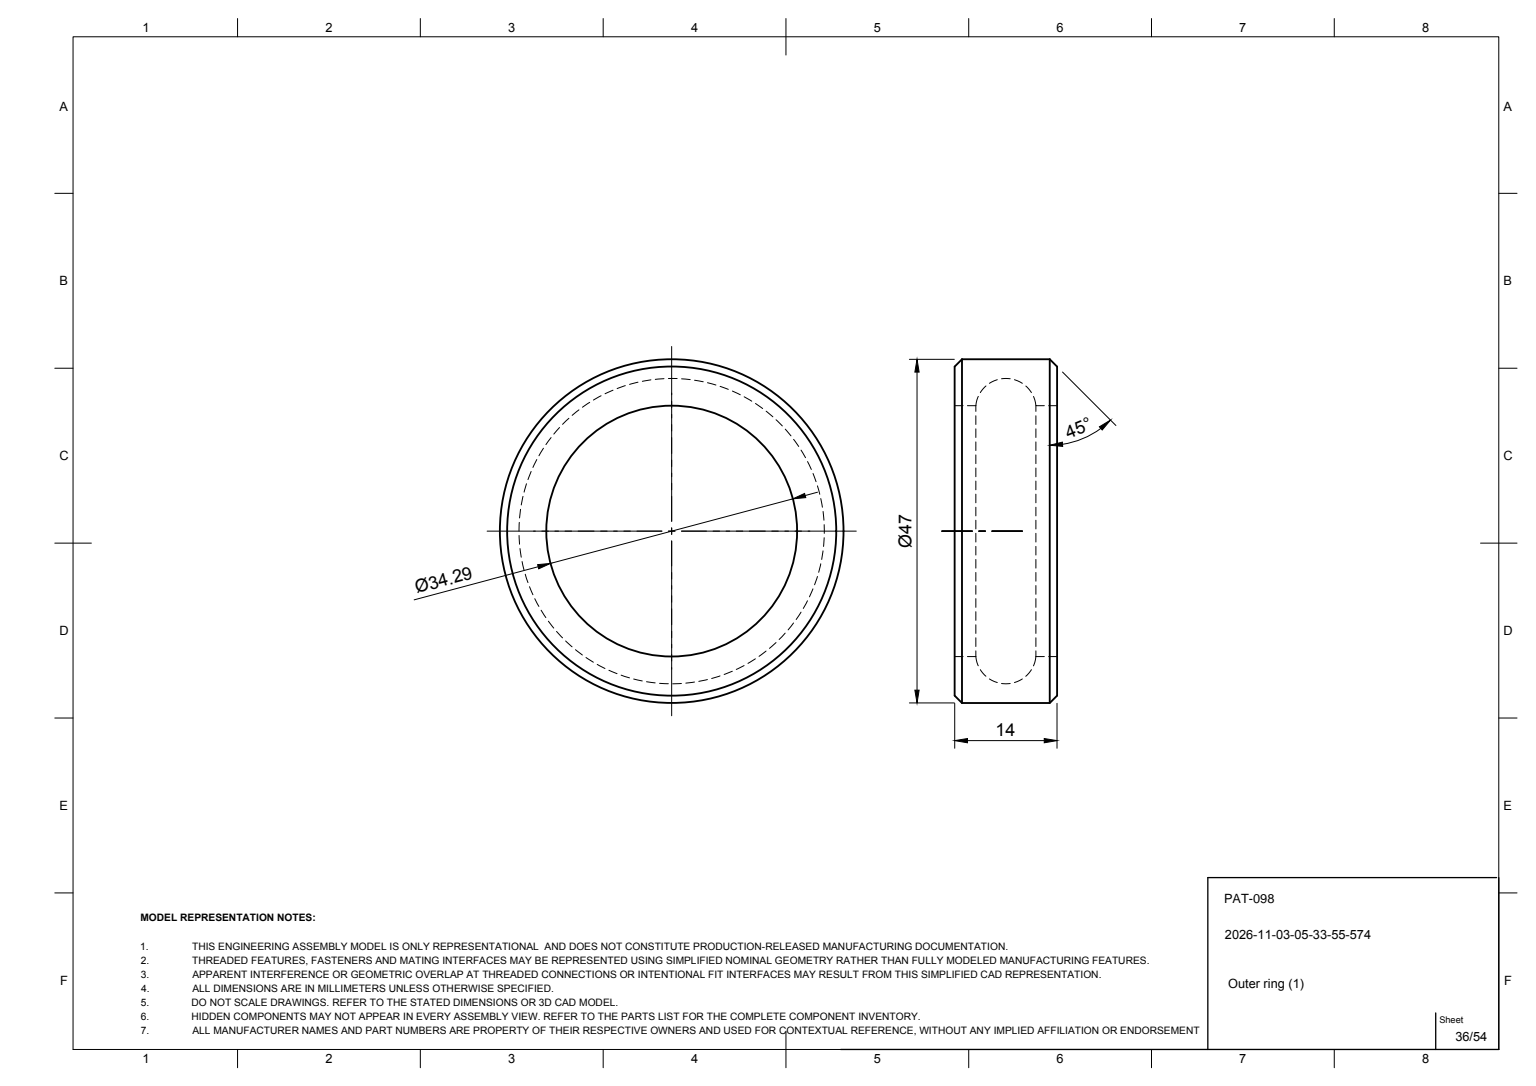
ISO-10303-21;
HEADER;
/* Generated by software containing ST-Developer
 * from STEP Tools, Inc. (www.steptools.com) 
 */

FILE_DESCRIPTION(
/* description */ ('Spring compression tester'),
/* implementation_level */ '2;1');

FILE_NAME(
/* name */ 'Outer ring (1).step',
/* time_stamp */ '2026-10-28T03:24:11-07:00',
/* author */ (''),
/* organization */ (''),
/* preprocessor_version */ 'ST-DEVELOPER v20.2',
/* originating_system */ 'Autodesk Translation Framework v15.17.0.0',
/* authorisation */ '');

FILE_SCHEMA (('AUTOMOTIVE_DESIGN { 1 0 10303 214 3 1 1 }'));
ENDSEC;

DATA;
#10=MECHANICAL_DESIGN_GEOMETRIC_PRESENTATION_REPRESENTATION('',(#1140),#43521);
#930=TOROIDAL_SURFACE('',#20142,1.675,0.412776);
#956=CONICAL_SURFACE('',#20153,2.3,0.785398163397449);
#957=CONICAL_SURFACE('',#20157,2.3,0.785398163397449);
#1013=SHAPE_REPRESENTATION_RELATIONSHIP('SRR','None',#43827,#1073);
#1073=ADVANCED_BREP_SHAPE_REPRESENTATION('',(#1214),#43487);
#1140=STYLED_ITEM('',(#44202),#1214);
#1214=MANIFOLD_SOLID_BREP('Body1',#18578);
#1461=FACE_BOUND('',#3916,.T.);
#1462=FACE_BOUND('',#3921,.T.);
#1906=PLANE('',#20150);
#1907=PLANE('',#20159);
#2652=FACE_OUTER_BOUND('',#3913,.T.);
#2653=FACE_OUTER_BOUND('',#3914,.T.);
#2654=FACE_OUTER_BOUND('',#3915,.T.);
#2655=FACE_OUTER_BOUND('',#3917,.T.);
#2656=FACE_OUTER_BOUND('',#3918,.T.);
#2657=FACE_OUTER_BOUND('',#3919,.T.);
#2658=FACE_OUTER_BOUND('',#3920,.T.);
#2659=FACE_OUTER_BOUND('',#3922,.T.);
#3913=EDGE_LOOP('',(#14351,#14352,#14353,#14354,#14355,#14356));
#3914=EDGE_LOOP('',(#14357,#14358,#14359,#14360,#14361));
#3915=EDGE_LOOP('',(#14362));
#3916=EDGE_LOOP('',(#14363));
#3917=EDGE_LOOP('',(#14364,#14365,#14366,#14367));
#3918=EDGE_LOOP('',(#14368,#14369,#14370,#14371));
#3919=EDGE_LOOP('',(#14372,#14373,#14374,#14375));
#3920=EDGE_LOOP('',(#14376));
#3921=EDGE_LOOP('',(#14377));
#3922=EDGE_LOOP('',(#14378,#14379,#14380,#14381,#14382));
#5322=LINE('',#29064,#6754);
#5323=LINE('',#29073,#6755);
#5324=LINE('',#29077,#6756);
#5325=LINE('',#29081,#6757);
#5326=LINE('',#29084,#6758);
#6754=VECTOR('',#23644,1.71469);
#6755=VECTOR('',#23655,2.3);
#6756=VECTOR('',#23660,2.35);
#6757=VECTOR('',#23665,2.3);
#6758=VECTOR('',#23670,1.71469);
#7807=CIRCLE('',#20143,1.71469);
#7808=CIRCLE('',#20144,1.71469);
#7809=CIRCLE('',#20145,0.412776);
#7810=CIRCLE('',#20146,1.71469);
#7811=CIRCLE('',#20147,1.71469);
#7812=CIRCLE('',#20149,1.71469);
#7813=CIRCLE('',#20151,2.25);
#7814=CIRCLE('',#20152,1.71469);
#7815=CIRCLE('',#20154,2.35);
#7816=CIRCLE('',#20156,2.35);
#7817=CIRCLE('',#20158,2.25);
#8853=VERTEX_POINT('',#29052);
#8854=VERTEX_POINT('',#29053);
#8855=VERTEX_POINT('',#29056);
#8856=VERTEX_POINT('',#29058);
#8857=VERTEX_POINT('',#29062);
#8858=VERTEX_POINT('',#29066);
#8859=VERTEX_POINT('',#29068);
#8860=VERTEX_POINT('',#29071);
#8861=VERTEX_POINT('',#29075);
#8862=VERTEX_POINT('',#29079);
#10840=EDGE_CURVE('',#8853,#8854,#7807,.T.);
#10841=EDGE_CURVE('',#8854,#8853,#7808,.T.);
#10842=EDGE_CURVE('',#8854,#8855,#7809,.T.);
#10843=EDGE_CURVE('',#8856,#8855,#7810,.T.);
#10844=EDGE_CURVE('',#8855,#8856,#7811,.T.);
#10845=EDGE_CURVE('',#8857,#8857,#7812,.T.);
#10846=EDGE_CURVE('',#8857,#8856,#5322,.T.);
#10847=EDGE_CURVE('',#8858,#8858,#7813,.T.);
#10848=EDGE_CURVE('',#8859,#8859,#7814,.T.);
#10849=EDGE_CURVE('',#8860,#8860,#7815,.T.);
#10850=EDGE_CURVE('',#8860,#8858,#5323,.T.);
#10851=EDGE_CURVE('',#8861,#8861,#7816,.T.);
#10852=EDGE_CURVE('',#8861,#8860,#5324,.T.);
#10853=EDGE_CURVE('',#8862,#8862,#7817,.T.);
#10854=EDGE_CURVE('',#8862,#8861,#5325,.T.);
#10855=EDGE_CURVE('',#8853,#8859,#5326,.T.);
#14351=ORIENTED_EDGE('',*,*,#10840,.F.);
#14352=ORIENTED_EDGE('',*,*,#10841,.F.);
#14353=ORIENTED_EDGE('',*,*,#10842,.T.);
#14354=ORIENTED_EDGE('',*,*,#10843,.F.);
#14355=ORIENTED_EDGE('',*,*,#10844,.F.);
#14356=ORIENTED_EDGE('',*,*,#10842,.F.);
#14357=ORIENTED_EDGE('',*,*,#10845,.T.);
#14358=ORIENTED_EDGE('',*,*,#10846,.T.);
#14359=ORIENTED_EDGE('',*,*,#10843,.T.);
#14360=ORIENTED_EDGE('',*,*,#10844,.T.);
#14361=ORIENTED_EDGE('',*,*,#10846,.F.);
#14362=ORIENTED_EDGE('',*,*,#10847,.F.);
#14363=ORIENTED_EDGE('',*,*,#10848,.T.);
#14364=ORIENTED_EDGE('',*,*,#10849,.F.);
#14365=ORIENTED_EDGE('',*,*,#10850,.T.);
#14366=ORIENTED_EDGE('',*,*,#10847,.T.);
#14367=ORIENTED_EDGE('',*,*,#10850,.F.);
#14368=ORIENTED_EDGE('',*,*,#10851,.F.);
#14369=ORIENTED_EDGE('',*,*,#10852,.T.);
#14370=ORIENTED_EDGE('',*,*,#10849,.T.);
#14371=ORIENTED_EDGE('',*,*,#10852,.F.);
#14372=ORIENTED_EDGE('',*,*,#10853,.F.);
#14373=ORIENTED_EDGE('',*,*,#10854,.T.);
#14374=ORIENTED_EDGE('',*,*,#10851,.T.);
#14375=ORIENTED_EDGE('',*,*,#10854,.F.);
#14376=ORIENTED_EDGE('',*,*,#10853,.T.);
#14377=ORIENTED_EDGE('',*,*,#10845,.F.);
#14378=ORIENTED_EDGE('',*,*,#10840,.T.);
#14379=ORIENTED_EDGE('',*,*,#10841,.T.);
#14380=ORIENTED_EDGE('',*,*,#10855,.T.);
#14381=ORIENTED_EDGE('',*,*,#10848,.F.);
#14382=ORIENTED_EDGE('',*,*,#10855,.F.);
#17242=CYLINDRICAL_SURFACE('',#20148,1.71469);
#17243=CYLINDRICAL_SURFACE('',#20155,2.35);
#17244=CYLINDRICAL_SURFACE('',#20160,1.71469);
#17976=ADVANCED_FACE('',(#2652),#930,.F.);
#17977=ADVANCED_FACE('',(#2653),#17242,.F.);
#17978=ADVANCED_FACE('',(#2654,#1461),#1906,.T.);
#17979=ADVANCED_FACE('',(#2655),#956,.T.);
#17980=ADVANCED_FACE('',(#2656),#17243,.T.);
#17981=ADVANCED_FACE('',(#2657),#957,.T.);
#17982=ADVANCED_FACE('',(#2658,#1462),#1907,.T.);
#17983=ADVANCED_FACE('',(#2659),#17244,.F.);
#18578=CLOSED_SHELL('',(#17976,#17977,#17978,#17979,#17980,#17981,#17982,
#17983));
#20141=AXIS2_PLACEMENT_3D('',#29050,#23626,#23627);
#20142=AXIS2_PLACEMENT_3D('',#29051,#23628,#23629);
#20143=AXIS2_PLACEMENT_3D('',#29054,#23630,#23631);
#20144=AXIS2_PLACEMENT_3D('',#29055,#23632,#23633);
#20145=AXIS2_PLACEMENT_3D('',#29057,#23634,#23635);
#20146=AXIS2_PLACEMENT_3D('',#29059,#23636,#23637);
#20147=AXIS2_PLACEMENT_3D('',#29060,#23638,#23639);
#20148=AXIS2_PLACEMENT_3D('',#29061,#23640,#23641);
#20149=AXIS2_PLACEMENT_3D('',#29063,#23642,#23643);
#20150=AXIS2_PLACEMENT_3D('',#29065,#23645,#23646);
#20151=AXIS2_PLACEMENT_3D('',#29067,#23647,#23648);
#20152=AXIS2_PLACEMENT_3D('',#29069,#23649,#23650);
#20153=AXIS2_PLACEMENT_3D('',#29070,#23651,#23652);
#20154=AXIS2_PLACEMENT_3D('',#29072,#23653,#23654);
#20155=AXIS2_PLACEMENT_3D('',#29074,#23656,#23657);
#20156=AXIS2_PLACEMENT_3D('',#29076,#23658,#23659);
#20157=AXIS2_PLACEMENT_3D('',#29078,#23661,#23662);
#20158=AXIS2_PLACEMENT_3D('',#29080,#23663,#23664);
#20159=AXIS2_PLACEMENT_3D('',#29082,#23666,#23667);
#20160=AXIS2_PLACEMENT_3D('',#29083,#23668,#23669);
#23626=DIRECTION('axis',(0.,0.,1.));
#23627=DIRECTION('refdir',(1.,0.,0.));
#23628=DIRECTION('center_axis',(0.,-1.,0.));
#23629=DIRECTION('ref_axis',(0.,0.,-1.));
#23630=DIRECTION('center_axis',(0.,-1.,0.));
#23631=DIRECTION('ref_axis',(1.,0.,0.));
#23632=DIRECTION('center_axis',(0.,-1.,0.));
#23633=DIRECTION('ref_axis',(1.,0.,0.));
#23634=DIRECTION('center_axis',(1.,0.,1.22464679914735E-16));
#23635=DIRECTION('ref_axis',(-1.22464679914735E-16,0.,1.));
#23636=DIRECTION('center_axis',(0.,1.,0.));
#23637=DIRECTION('ref_axis',(1.,0.,0.));
#23638=DIRECTION('center_axis',(0.,1.,0.));
#23639=DIRECTION('ref_axis',(1.,0.,0.));
#23640=DIRECTION('center_axis',(0.,-1.,0.));
#23641=DIRECTION('ref_axis',(1.,0.,0.));
#23642=DIRECTION('center_axis',(0.,-1.,0.));
#23643=DIRECTION('ref_axis',(1.,0.,0.));
#23644=DIRECTION('',(0.,1.,0.));
#23645=DIRECTION('center_axis',(0.,1.,0.));
#23646=DIRECTION('ref_axis',(0.,0.,1.));
#23647=DIRECTION('center_axis',(0.,-1.,0.));
#23648=DIRECTION('ref_axis',(1.,0.,0.));
#23649=DIRECTION('center_axis',(0.,-1.,0.));
#23650=DIRECTION('ref_axis',(1.,0.,0.));
#23651=DIRECTION('center_axis',(0.,-1.,0.));
#23652=DIRECTION('ref_axis',(1.,0.,0.));
#23653=DIRECTION('center_axis',(0.,-1.,0.));
#23654=DIRECTION('ref_axis',(1.,0.,0.));
#23655=DIRECTION('',(0.707106781186548,0.707106781186547,8.65956056235494E-17));
#23656=DIRECTION('center_axis',(0.,-1.,0.));
#23657=DIRECTION('ref_axis',(1.,0.,0.));
#23658=DIRECTION('center_axis',(0.,-1.,0.));
#23659=DIRECTION('ref_axis',(1.,0.,0.));
#23660=DIRECTION('',(0.,1.,0.));
#23661=DIRECTION('center_axis',(0.,1.,0.));
#23662=DIRECTION('ref_axis',(1.,0.,0.));
#23663=DIRECTION('center_axis',(0.,-1.,0.));
#23664=DIRECTION('ref_axis',(1.,0.,0.));
#23665=DIRECTION('',(-0.707106781186548,0.707106781186547,-8.65956056235494E-17));
#23666=DIRECTION('center_axis',(0.,-1.,0.));
#23667=DIRECTION('ref_axis',(0.,0.,-1.));
#23668=DIRECTION('center_axis',(0.,-1.,0.));
#23669=DIRECTION('ref_axis',(1.,0.,0.));
#23670=DIRECTION('',(0.,1.,0.));
#29050=CARTESIAN_POINT('',(0.,0.,0.));
#29051=CARTESIAN_POINT('Origin',(0.,0.,0.));
#29052=CARTESIAN_POINT('',(-1.71469,0.410863395882378,-2.09988962002998E-16));
#29053=CARTESIAN_POINT('',(-2.09988962002998E-16,0.410863395882378,1.71469));
#29054=CARTESIAN_POINT('Origin',(0.,0.410863395882378,0.));
#29055=CARTESIAN_POINT('Origin',(0.,0.410863395882378,0.));
#29056=CARTESIAN_POINT('',(-2.09988962002998E-16,-0.410863395882378,1.71469));
#29057=CARTESIAN_POINT('Origin',(-2.05128338857182E-16,0.,1.675));
#29058=CARTESIAN_POINT('',(-1.71469,-0.410863395882378,2.09988962002998E-16));
#29059=CARTESIAN_POINT('Origin',(0.,-0.410863395882378,0.));
#29060=CARTESIAN_POINT('Origin',(0.,-0.410863395882378,0.));
#29061=CARTESIAN_POINT('Origin',(0.,0.,0.));
#29062=CARTESIAN_POINT('',(-1.71469,-0.7,-2.09988962002998E-16));
#29063=CARTESIAN_POINT('Origin',(0.,-0.7,0.));
#29064=CARTESIAN_POINT('',(-1.71469,0.,-2.09988962002998E-16));
#29065=CARTESIAN_POINT('Origin',(2.25,0.7,0.));
#29066=CARTESIAN_POINT('',(-2.25,0.7,-2.75545529808154E-16));
#29067=CARTESIAN_POINT('Origin',(0.,0.7,0.));
#29068=CARTESIAN_POINT('',(-1.71469,0.7,-2.09988962002998E-16));
#29069=CARTESIAN_POINT('Origin',(0.,0.7,0.));
#29070=CARTESIAN_POINT('Origin',(0.,0.65,0.));
#29071=CARTESIAN_POINT('',(-2.35,0.6,-2.87791997799628E-16));
#29072=CARTESIAN_POINT('Origin',(0.,0.6,0.));
#29073=CARTESIAN_POINT('',(-2.3,0.65,-2.81668763803891E-16));
#29074=CARTESIAN_POINT('Origin',(0.,0.,0.));
#29075=CARTESIAN_POINT('',(-2.35,-0.6,-2.87791997799628E-16));
#29076=CARTESIAN_POINT('Origin',(0.,-0.6,0.));
#29077=CARTESIAN_POINT('',(-2.35,0.,-2.87791997799628E-16));
#29078=CARTESIAN_POINT('Origin',(0.,-0.65,0.));
#29079=CARTESIAN_POINT('',(-2.25,-0.7,-2.75545529808154E-16));
#29080=CARTESIAN_POINT('Origin',(0.,-0.7,0.));
#29081=CARTESIAN_POINT('',(-2.3,-0.65,-2.81668763803891E-16));
#29082=CARTESIAN_POINT('Origin',(1.71469,-0.7,0.));
#29083=CARTESIAN_POINT('Origin',(0.,0.,0.));
#29084=CARTESIAN_POINT('',(-1.71469,0.,-2.09988962002998E-16));
#43419=UNCERTAINTY_MEASURE_WITH_UNIT(LENGTH_MEASURE(0.001),#43522,
'DISTANCE_ACCURACY_VALUE',
'Maximum model space distance between geometric entities at asserted c
onnectivities');
#43453=UNCERTAINTY_MEASURE_WITH_UNIT(LENGTH_MEASURE(0.001),#43522,
'DISTANCE_ACCURACY_VALUE',
'Maximum model space distance between geometric entities at asserted c
onnectivities');
#43487=(
GEOMETRIC_REPRESENTATION_CONTEXT(3)
GLOBAL_UNCERTAINTY_ASSIGNED_CONTEXT((#43419))
GLOBAL_UNIT_ASSIGNED_CONTEXT((#43522,#43524,#43525))
REPRESENTATION_CONTEXT('','3D')
);
#43521=(
GEOMETRIC_REPRESENTATION_CONTEXT(3)
GLOBAL_UNCERTAINTY_ASSIGNED_CONTEXT((#43453))
GLOBAL_UNIT_ASSIGNED_CONTEXT((#43522,#43524,#43525))
REPRESENTATION_CONTEXT('','3D')
);
#43522=(
LENGTH_UNIT()
NAMED_UNIT(*)
SI_UNIT(.CENTI.,.METRE.)
);
#43524=(
NAMED_UNIT(*)
PLANE_ANGLE_UNIT()
SI_UNIT($,.RADIAN.)
);
#43525=(
NAMED_UNIT(*)
SI_UNIT($,.STERADIAN.)
SOLID_ANGLE_UNIT()
);
#43559=SHAPE_DEFINITION_REPRESENTATION(#43631,#43827);
#43631=PRODUCT_DEFINITION_SHAPE('',$,#43895);
#43827=SHAPE_REPRESENTATION('',(#20141),#43487);
#43861=PRODUCT_DEFINITION_CONTEXT('part definition',#44064,'design');
#43895=PRODUCT_DEFINITION('Outer ring (1)','Outer ring (1)',#43962,#43861);
#43962=PRODUCT_DEFINITION_FORMATION('',$,#44099);
#44064=APPLICATION_CONTEXT(
'Core Data for Automotive Mechanical Design Process');
#44065=PRODUCT_CONTEXT('part definition',#44064,'mechanical');
#44099=PRODUCT('Outer ring (1)','Outer ring (1)','Outer ring (1)',(#44065));
#44196=COLOUR_RGB('Grey',0.48,0.52,0.57);
#44197=FILL_AREA_STYLE_COLOUR('',#44196);
#44198=FILL_AREA_STYLE('',(#44197));
#44199=SURFACE_STYLE_FILL_AREA(#44198);
#44200=SURFACE_SIDE_STYLE('',(#44199));
#44201=SURFACE_STYLE_USAGE(.BOTH.,#44200);
#44202=PRESENTATION_STYLE_ASSIGNMENT((#44201));
ENDSEC;
END-ISO-10303-21;
